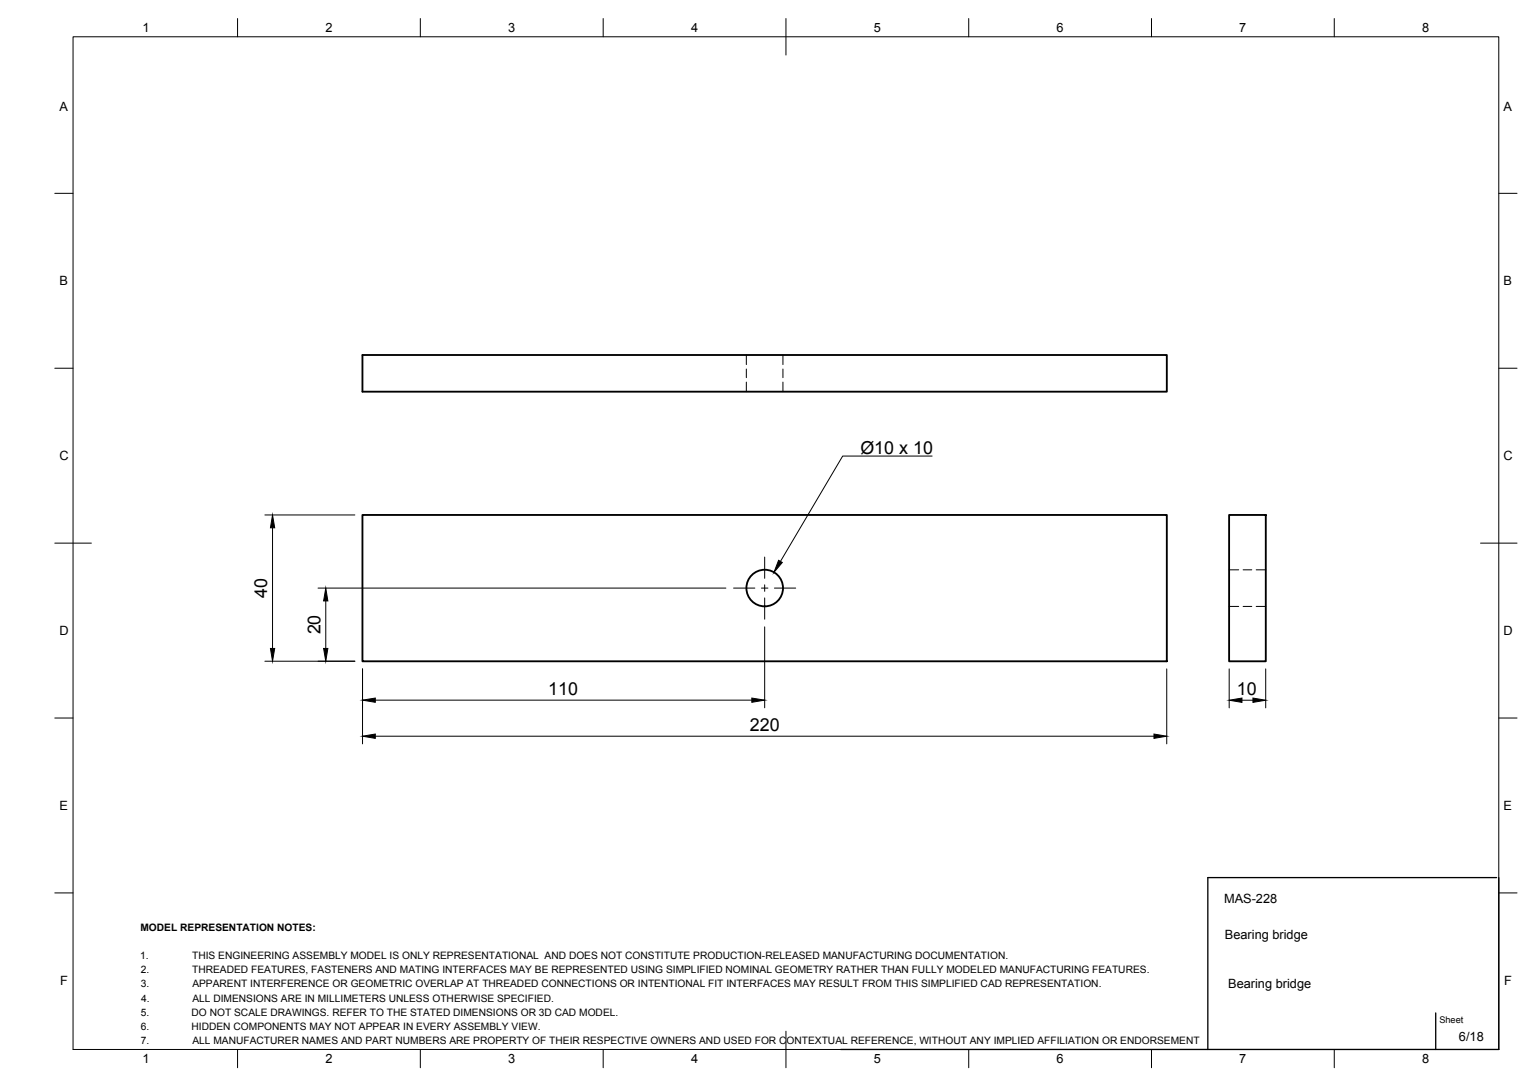
ISO-10303-21;
HEADER;
/* Generated by software containing ST-Developer
 * from STEP Tools, Inc. (www.steptools.com) 
 */

FILE_DESCRIPTION(
/* description */ ('Independent Peaucellier-Lipkin straight-line linkage. Radius arms 100
 mm, inversion-cell links 60 mm, crank radius and fixed-pivot spacing 
32 mm. Inversion constant 6400 mm squared, nominal output straight lin
e X=100 mm. Overhead bearing bridge clears the layered moving links. N
o accuracy or load rating assigned.'),
/* implementation_level */ '2;1');

FILE_NAME(
/* name */ 'Bearing bridge.step',
/* time_stamp */ '2026-11-09T18:06:16-08:00',
/* author */ (''),
/* organization */ (''),
/* preprocessor_version */ 'ST-DEVELOPER v20.2',
/* originating_system */ 'Autodesk Translation Framework v15.17.0.0',
/* authorisation */ '');

FILE_SCHEMA (('AUTOMOTIVE_DESIGN { 1 0 10303 214 3 1 1 }'));
ENDSEC;

DATA;
#10=MECHANICAL_DESIGN_GEOMETRIC_PRESENTATION_REPRESENTATION('',(#284),#3581);
#250=SHAPE_REPRESENTATION_RELATIONSHIP('SRR','None',#3684,#267);
#267=ADVANCED_BREP_SHAPE_REPRESENTATION('',(#301),#3566);
#284=STYLED_ITEM('',(#3778),#301);
#301=MANIFOLD_SOLID_BREP('Body1',#1870);
#328=FACE_BOUND('',#569,.T.);
#329=FACE_BOUND('',#571,.T.);
#372=PLANE('',#2109);
#373=PLANE('',#2110);
#374=PLANE('',#2111);
#375=PLANE('',#2112);
#376=PLANE('',#2113);
#377=PLANE('',#2114);
#440=FACE_OUTER_BOUND('',#563,.T.);
#441=FACE_OUTER_BOUND('',#564,.T.);
#442=FACE_OUTER_BOUND('',#565,.T.);
#443=FACE_OUTER_BOUND('',#566,.T.);
#444=FACE_OUTER_BOUND('',#567,.T.);
#445=FACE_OUTER_BOUND('',#568,.T.);
#446=FACE_OUTER_BOUND('',#570,.T.);
#563=EDGE_LOOP('',(#1382,#1383,#1384,#1385));
#564=EDGE_LOOP('',(#1386,#1387,#1388,#1389));
#565=EDGE_LOOP('',(#1390,#1391,#1392,#1393));
#566=EDGE_LOOP('',(#1394,#1395,#1396,#1397));
#567=EDGE_LOOP('',(#1398,#1399,#1400,#1401));
#568=EDGE_LOOP('',(#1402,#1403,#1404,#1405));
#569=EDGE_LOOP('',(#1406));
#570=EDGE_LOOP('',(#1407,#1408,#1409,#1410));
#571=EDGE_LOOP('',(#1411));
#714=LINE('',#3107,#812);
#715=LINE('',#3112,#813);
#716=LINE('',#3114,#814);
#717=LINE('',#3116,#815);
#718=LINE('',#3117,#816);
#719=LINE('',#3120,#817);
#720=LINE('',#3122,#818);
#721=LINE('',#3123,#819);
#722=LINE('',#3126,#820);
#723=LINE('',#3128,#821);
#724=LINE('',#3129,#822);
#725=LINE('',#3131,#823);
#726=LINE('',#3132,#824);
#812=VECTOR('',#2448,5.);
#813=VECTOR('',#2453,10.);
#814=VECTOR('',#2454,10.);
#815=VECTOR('',#2455,10.);
#816=VECTOR('',#2456,10.);
#817=VECTOR('',#2459,10.);
#818=VECTOR('',#2460,10.);
#819=VECTOR('',#2461,10.);
#820=VECTOR('',#2464,10.);
#821=VECTOR('',#2465,10.);
#822=VECTOR('',#2466,10.);
#823=VECTOR('',#2469,10.);
#824=VECTOR('',#2470,10.);
#905=CIRCLE('',#2107,5.);
#906=CIRCLE('',#2108,5.);
#1011=VERTEX_POINT('',#3104);
#1012=VERTEX_POINT('',#3106);
#1013=VERTEX_POINT('',#3110);
#1014=VERTEX_POINT('',#3111);
#1015=VERTEX_POINT('',#3113);
#1016=VERTEX_POINT('',#3115);
#1017=VERTEX_POINT('',#3119);
#1018=VERTEX_POINT('',#3121);
#1019=VERTEX_POINT('',#3125);
#1020=VERTEX_POINT('',#3127);
#1153=EDGE_CURVE('',#1011,#1011,#905,.T.);
#1154=EDGE_CURVE('',#1011,#1012,#714,.T.);
#1155=EDGE_CURVE('',#1012,#1012,#906,.T.);
#1156=EDGE_CURVE('',#1013,#1014,#715,.T.);
#1157=EDGE_CURVE('',#1014,#1015,#716,.T.);
#1158=EDGE_CURVE('',#1016,#1015,#717,.T.);
#1159=EDGE_CURVE('',#1013,#1016,#718,.T.);
#1160=EDGE_CURVE('',#1017,#1013,#719,.T.);
#1161=EDGE_CURVE('',#1018,#1016,#720,.T.);
#1162=EDGE_CURVE('',#1017,#1018,#721,.T.);
#1163=EDGE_CURVE('',#1019,#1017,#722,.T.);
#1164=EDGE_CURVE('',#1020,#1018,#723,.T.);
#1165=EDGE_CURVE('',#1019,#1020,#724,.T.);
#1166=EDGE_CURVE('',#1014,#1019,#725,.T.);
#1167=EDGE_CURVE('',#1015,#1020,#726,.T.);
#1382=ORIENTED_EDGE('',*,*,#1153,.F.);
#1383=ORIENTED_EDGE('',*,*,#1154,.T.);
#1384=ORIENTED_EDGE('',*,*,#1155,.F.);
#1385=ORIENTED_EDGE('',*,*,#1154,.F.);
#1386=ORIENTED_EDGE('',*,*,#1156,.T.);
#1387=ORIENTED_EDGE('',*,*,#1157,.T.);
#1388=ORIENTED_EDGE('',*,*,#1158,.F.);
#1389=ORIENTED_EDGE('',*,*,#1159,.F.);
#1390=ORIENTED_EDGE('',*,*,#1160,.T.);
#1391=ORIENTED_EDGE('',*,*,#1159,.T.);
#1392=ORIENTED_EDGE('',*,*,#1161,.F.);
#1393=ORIENTED_EDGE('',*,*,#1162,.F.);
#1394=ORIENTED_EDGE('',*,*,#1163,.T.);
#1395=ORIENTED_EDGE('',*,*,#1162,.T.);
#1396=ORIENTED_EDGE('',*,*,#1164,.F.);
#1397=ORIENTED_EDGE('',*,*,#1165,.F.);
#1398=ORIENTED_EDGE('',*,*,#1166,.T.);
#1399=ORIENTED_EDGE('',*,*,#1165,.T.);
#1400=ORIENTED_EDGE('',*,*,#1167,.F.);
#1401=ORIENTED_EDGE('',*,*,#1157,.F.);
#1402=ORIENTED_EDGE('',*,*,#1167,.T.);
#1403=ORIENTED_EDGE('',*,*,#1164,.T.);
#1404=ORIENTED_EDGE('',*,*,#1161,.T.);
#1405=ORIENTED_EDGE('',*,*,#1158,.T.);
#1406=ORIENTED_EDGE('',*,*,#1153,.T.);
#1407=ORIENTED_EDGE('',*,*,#1166,.F.);
#1408=ORIENTED_EDGE('',*,*,#1156,.F.);
#1409=ORIENTED_EDGE('',*,*,#1160,.F.);
#1410=ORIENTED_EDGE('',*,*,#1163,.F.);
#1411=ORIENTED_EDGE('',*,*,#1155,.T.);
#1715=CYLINDRICAL_SURFACE('',#2106,5.);
#1772=ADVANCED_FACE('',(#440),#1715,.F.);
#1773=ADVANCED_FACE('',(#441),#372,.T.);
#1774=ADVANCED_FACE('',(#442),#373,.T.);
#1775=ADVANCED_FACE('',(#443),#374,.T.);
#1776=ADVANCED_FACE('',(#444),#375,.T.);
#1777=ADVANCED_FACE('',(#445,#328),#376,.T.);
#1778=ADVANCED_FACE('',(#446,#329),#377,.F.);
#1870=CLOSED_SHELL('',(#1772,#1773,#1774,#1775,#1776,#1777,#1778));
#2105=AXIS2_PLACEMENT_3D('',#3102,#2442,#2443);
#2106=AXIS2_PLACEMENT_3D('',#3103,#2444,#2445);
#2107=AXIS2_PLACEMENT_3D('',#3105,#2446,#2447);
#2108=AXIS2_PLACEMENT_3D('',#3108,#2449,#2450);
#2109=AXIS2_PLACEMENT_3D('',#3109,#2451,#2452);
#2110=AXIS2_PLACEMENT_3D('',#3118,#2457,#2458);
#2111=AXIS2_PLACEMENT_3D('',#3124,#2462,#2463);
#2112=AXIS2_PLACEMENT_3D('',#3130,#2467,#2468);
#2113=AXIS2_PLACEMENT_3D('',#3133,#2471,#2472);
#2114=AXIS2_PLACEMENT_3D('',#3134,#2473,#2474);
#2442=DIRECTION('axis',(0.,0.,1.));
#2443=DIRECTION('refdir',(1.,0.,0.));
#2444=DIRECTION('center_axis',(0.,0.,-1.));
#2445=DIRECTION('ref_axis',(1.,0.,0.));
#2446=DIRECTION('center_axis',(0.,0.,-1.));
#2447=DIRECTION('ref_axis',(1.,0.,0.));
#2448=DIRECTION('',(0.,0.,-1.));
#2449=DIRECTION('center_axis',(0.,0.,1.));
#2450=DIRECTION('ref_axis',(1.,0.,0.));
#2451=DIRECTION('center_axis',(0.,1.,0.));
#2452=DIRECTION('ref_axis',(-1.,0.,0.));
#2453=DIRECTION('',(-1.,0.,0.));
#2454=DIRECTION('',(0.,0.,1.));
#2455=DIRECTION('',(-1.,0.,0.));
#2456=DIRECTION('',(0.,0.,1.));
#2457=DIRECTION('center_axis',(1.,0.,0.));
#2458=DIRECTION('ref_axis',(0.,1.,0.));
#2459=DIRECTION('',(0.,1.,0.));
#2460=DIRECTION('',(0.,1.,0.));
#2461=DIRECTION('',(0.,0.,1.));
#2462=DIRECTION('center_axis',(0.,-1.,0.));
#2463=DIRECTION('ref_axis',(1.,0.,0.));
#2464=DIRECTION('',(1.,0.,0.));
#2465=DIRECTION('',(1.,0.,0.));
#2466=DIRECTION('',(0.,0.,1.));
#2467=DIRECTION('center_axis',(-1.,0.,0.));
#2468=DIRECTION('ref_axis',(0.,-1.,0.));
#2469=DIRECTION('',(0.,-1.,0.));
#2470=DIRECTION('',(0.,-1.,0.));
#2471=DIRECTION('center_axis',(0.,0.,1.));
#2472=DIRECTION('ref_axis',(1.,0.,0.));
#2473=DIRECTION('center_axis',(0.,0.,1.));
#2474=DIRECTION('ref_axis',(1.,0.,0.));
#3102=CARTESIAN_POINT('',(0.,0.,0.));
#3103=CARTESIAN_POINT('Origin',(32.,0.,5.));
#3104=CARTESIAN_POINT('',(27.,6.12323399573677E-16,10.));
#3105=CARTESIAN_POINT('Origin',(32.,0.,10.));
#3106=CARTESIAN_POINT('',(27.,6.12323399573677E-16,0.));
#3107=CARTESIAN_POINT('',(27.,6.12323399573677E-16,5.));
#3108=CARTESIAN_POINT('Origin',(32.,0.,0.));
#3109=CARTESIAN_POINT('Origin',(52.,110.,0.));
#3110=CARTESIAN_POINT('',(52.,110.,0.));
#3111=CARTESIAN_POINT('',(12.,110.,0.));
#3112=CARTESIAN_POINT('',(52.,110.,0.));
#3113=CARTESIAN_POINT('',(12.,110.,10.));
#3114=CARTESIAN_POINT('',(12.,110.,0.));
#3115=CARTESIAN_POINT('',(52.,110.,10.));
#3116=CARTESIAN_POINT('',(52.,110.,10.));
#3117=CARTESIAN_POINT('',(52.,110.,0.));
#3118=CARTESIAN_POINT('Origin',(52.,-110.,0.));
#3119=CARTESIAN_POINT('',(52.,-110.,0.));
#3120=CARTESIAN_POINT('',(52.,-110.,0.));
#3121=CARTESIAN_POINT('',(52.,-110.,10.));
#3122=CARTESIAN_POINT('',(52.,-110.,10.));
#3123=CARTESIAN_POINT('',(52.,-110.,0.));
#3124=CARTESIAN_POINT('Origin',(12.,-110.,0.));
#3125=CARTESIAN_POINT('',(12.,-110.,0.));
#3126=CARTESIAN_POINT('',(12.,-110.,0.));
#3127=CARTESIAN_POINT('',(12.,-110.,10.));
#3128=CARTESIAN_POINT('',(12.,-110.,10.));
#3129=CARTESIAN_POINT('',(12.,-110.,0.));
#3130=CARTESIAN_POINT('Origin',(12.,110.,0.));
#3131=CARTESIAN_POINT('',(12.,110.,0.));
#3132=CARTESIAN_POINT('',(12.,110.,10.));
#3133=CARTESIAN_POINT('Origin',(32.,0.,10.));
#3134=CARTESIAN_POINT('Origin',(32.,0.,0.));
#3547=UNCERTAINTY_MEASURE_WITH_UNIT(LENGTH_MEASURE(0.01),#3582,
'DISTANCE_ACCURACY_VALUE',
'Maximum model space distance between geometric entities at asserted c
onnectivities');
#3562=UNCERTAINTY_MEASURE_WITH_UNIT(LENGTH_MEASURE(0.01),#3582,
'DISTANCE_ACCURACY_VALUE',
'Maximum model space distance between geometric entities at asserted c
onnectivities');
#3566=(
GEOMETRIC_REPRESENTATION_CONTEXT(3)
GLOBAL_UNCERTAINTY_ASSIGNED_CONTEXT((#3547))
GLOBAL_UNIT_ASSIGNED_CONTEXT((#3582,#3584,#3585))
REPRESENTATION_CONTEXT('','3D')
);
#3581=(
GEOMETRIC_REPRESENTATION_CONTEXT(3)
GLOBAL_UNCERTAINTY_ASSIGNED_CONTEXT((#3562))
GLOBAL_UNIT_ASSIGNED_CONTEXT((#3582,#3584,#3585))
REPRESENTATION_CONTEXT('','3D')
);
#3582=(
LENGTH_UNIT()
NAMED_UNIT(*)
SI_UNIT(.MILLI.,.METRE.)
);
#3584=(
NAMED_UNIT(*)
PLANE_ANGLE_UNIT()
SI_UNIT($,.RADIAN.)
);
#3585=(
NAMED_UNIT(*)
SI_UNIT($,.STERADIAN.)
SOLID_ANGLE_UNIT()
);
#3589=SHAPE_DEFINITION_REPRESENTATION(#3607,#3684);
#3607=PRODUCT_DEFINITION_SHAPE('',$,#3703);
#3684=SHAPE_REPRESENTATION('',(#2105),#3566);
#3699=PRODUCT_DEFINITION_CONTEXT('part definition',#3755,'design');
#3703=PRODUCT_DEFINITION('Bearing bridge','Bearing bridge',#3721,#3699);
#3721=PRODUCT_DEFINITION_FORMATION('',$,#3760);
#3755=APPLICATION_CONTEXT(
'Core Data for Automotive Mechanical Design Process');
#3756=PRODUCT_CONTEXT('part definition',#3755,'mechanical');
#3760=PRODUCT('Bearing bridge','Bearing bridge',$,(#3756));
#3778=PRESENTATION_STYLE_ASSIGNMENT((#3791));
#3791=SURFACE_STYLE_USAGE(.BOTH.,#3804);
#3804=SURFACE_SIDE_STYLE('',(#3817));
#3817=SURFACE_STYLE_FILL_AREA(#3830);
#3830=FILL_AREA_STYLE('Dark blue',(#3843));
#3843=FILL_AREA_STYLE_COLOUR('Dark blue',#3856);
#3856=COLOUR_RGB('Dark blue',0.0901960784313725,0.270588235294118,0.513725490196078);
ENDSEC;
END-ISO-10303-21;
